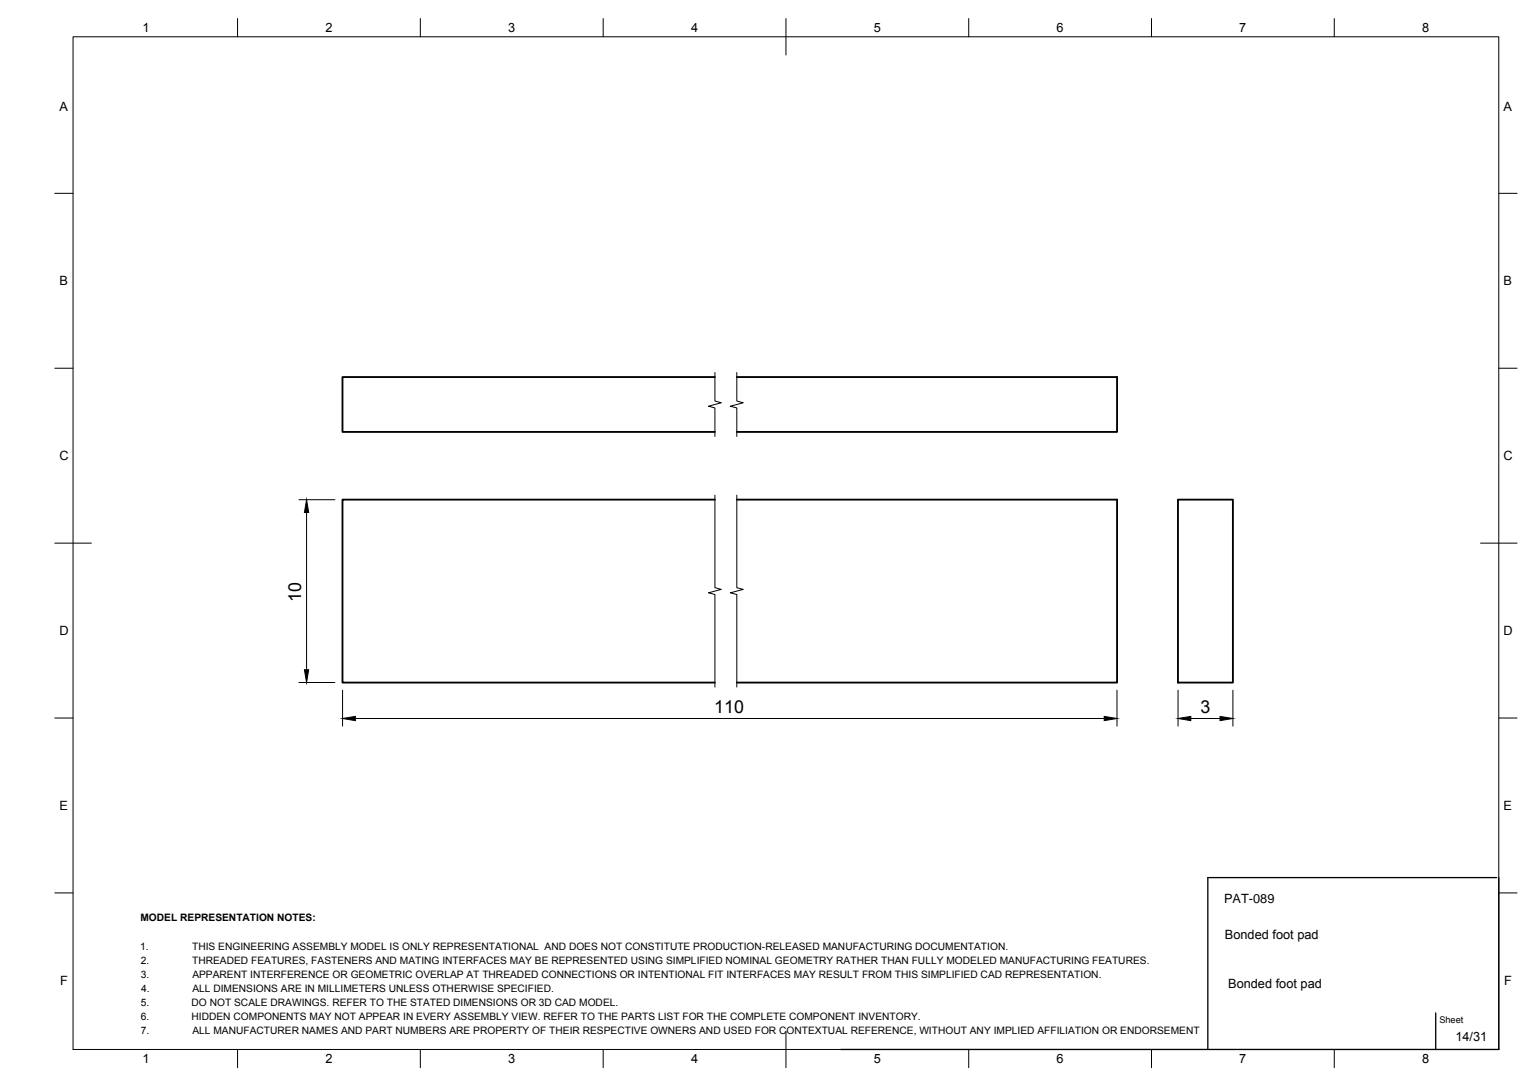
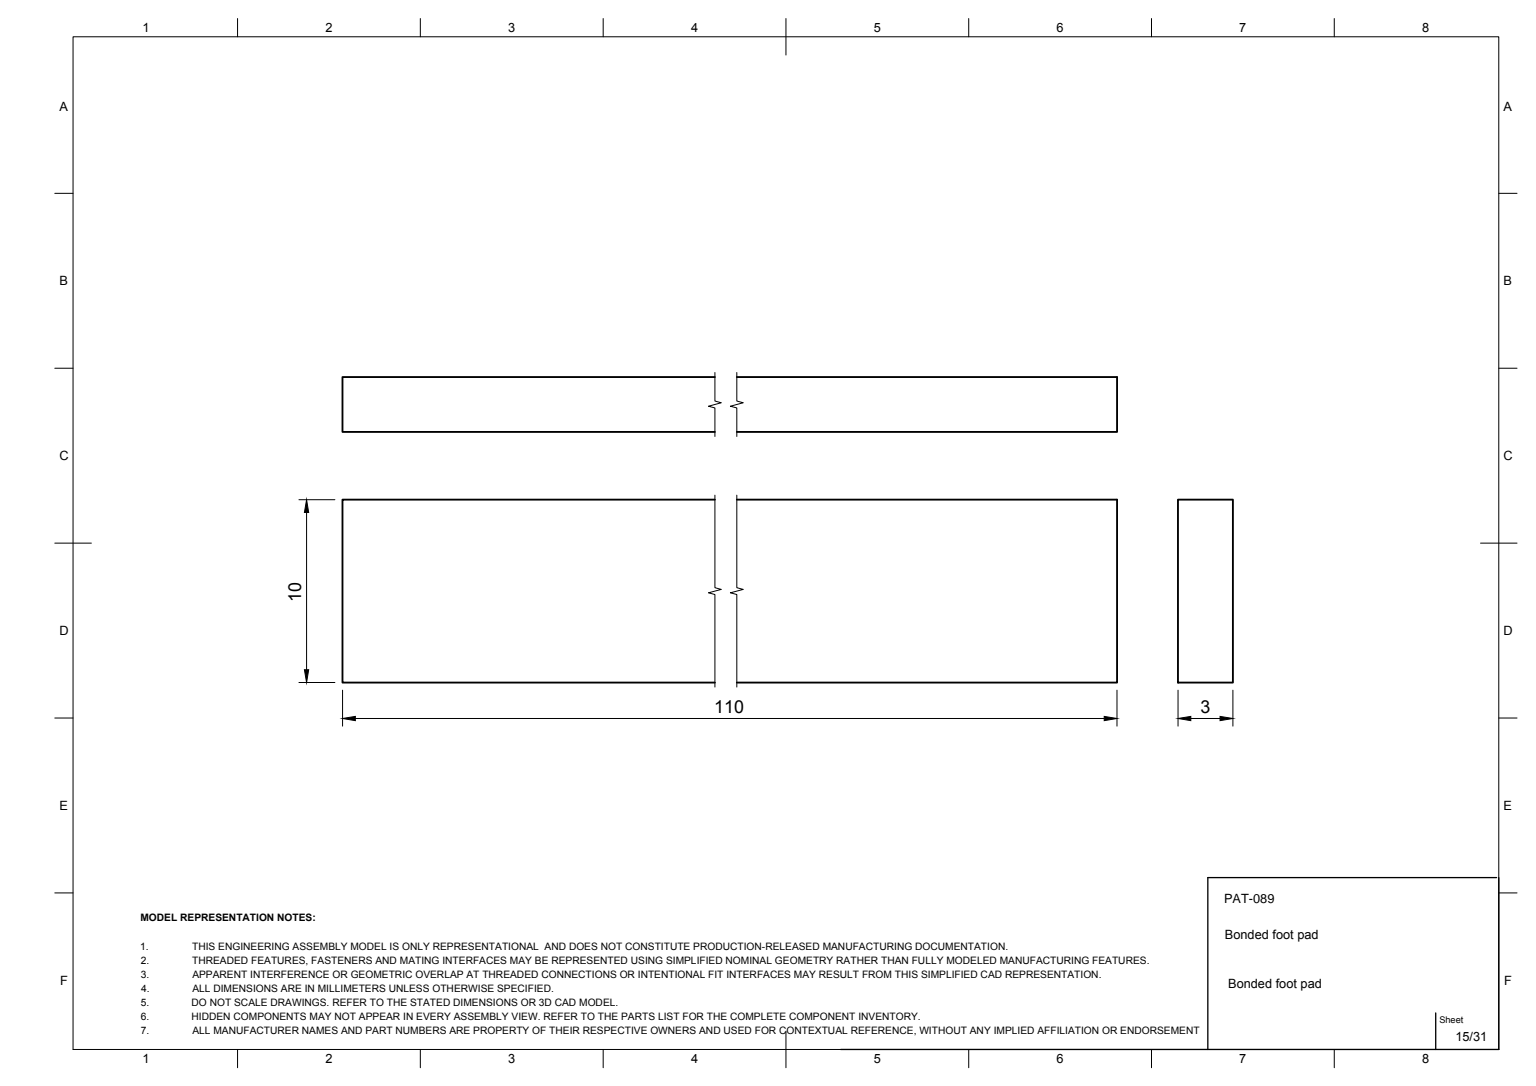
ISO-10303-21;
HEADER;
/* Generated by software containing ST-Developer
 * from STEP Tools, Inc. (www.steptools.com) 
 */

FILE_DESCRIPTION(
/* description */ ('Rotary union on bearing shaft'),
/* implementation_level */ '2;1');

FILE_NAME(
/* name */ 'Bonded foot pad.step',
/* time_stamp */ '2026-10-28T03:24:01-07:00',
/* author */ (''),
/* organization */ (''),
/* preprocessor_version */ 'ST-DEVELOPER v20.2',
/* originating_system */ 'Autodesk Translation Framework v15.17.0.0',
/* authorisation */ '');

FILE_SCHEMA (('AUTOMOTIVE_DESIGN { 1 0 10303 214 3 1 1 }'));
ENDSEC;

DATA;
#10=MECHANICAL_DESIGN_GEOMETRIC_PRESENTATION_REPRESENTATION('',(#322),#9448);
#268=SHAPE_REPRESENTATION_RELATIONSHIP('SRR','None',#9568,#295);
#295=ADVANCED_BREP_SHAPE_REPRESENTATION('',(#357),#9428);
#322=STYLED_ITEM('',(#9771),#357);
#357=MANIFOLD_SOLID_BREP('Body1',#4877);
#538=PLANE('',#5414);
#539=PLANE('',#5415);
#540=PLANE('',#5416);
#541=PLANE('',#5417);
#542=PLANE('',#5418);
#543=PLANE('',#5419);
#755=FACE_OUTER_BOUND('',#1118,.T.);
#756=FACE_OUTER_BOUND('',#1119,.T.);
#757=FACE_OUTER_BOUND('',#1120,.T.);
#758=FACE_OUTER_BOUND('',#1121,.T.);
#759=FACE_OUTER_BOUND('',#1122,.T.);
#760=FACE_OUTER_BOUND('',#1123,.T.);
#1118=EDGE_LOOP('',(#3675,#3676,#3677,#3678));
#1119=EDGE_LOOP('',(#3679,#3680,#3681,#3682));
#1120=EDGE_LOOP('',(#3683,#3684,#3685,#3686));
#1121=EDGE_LOOP('',(#3687,#3688,#3689,#3690));
#1122=EDGE_LOOP('',(#3691,#3692,#3693,#3694));
#1123=EDGE_LOOP('',(#3695,#3696,#3697,#3698));
#1458=LINE('',#7978,#1778);
#1459=LINE('',#7980,#1779);
#1460=LINE('',#7982,#1780);
#1461=LINE('',#7983,#1781);
#1462=LINE('',#7986,#1782);
#1463=LINE('',#7988,#1783);
#1464=LINE('',#7989,#1784);
#1465=LINE('',#7992,#1785);
#1466=LINE('',#7994,#1786);
#1467=LINE('',#7995,#1787);
#1468=LINE('',#7997,#1788);
#1469=LINE('',#7998,#1789);
#1778=VECTOR('',#6347,1.);
#1779=VECTOR('',#6348,1.);
#1780=VECTOR('',#6349,1.);
#1781=VECTOR('',#6350,1.);
#1782=VECTOR('',#6353,1.);
#1783=VECTOR('',#6354,1.);
#1784=VECTOR('',#6355,1.);
#1785=VECTOR('',#6358,1.);
#1786=VECTOR('',#6359,1.);
#1787=VECTOR('',#6360,1.);
#1788=VECTOR('',#6363,1.);
#1789=VECTOR('',#6364,1.);
#2388=VERTEX_POINT('',#7976);
#2389=VERTEX_POINT('',#7977);
#2390=VERTEX_POINT('',#7979);
#2391=VERTEX_POINT('',#7981);
#2392=VERTEX_POINT('',#7985);
#2393=VERTEX_POINT('',#7987);
#2394=VERTEX_POINT('',#7991);
#2395=VERTEX_POINT('',#7993);
#2865=EDGE_CURVE('',#2388,#2389,#1458,.T.);
#2866=EDGE_CURVE('',#2389,#2390,#1459,.T.);
#2867=EDGE_CURVE('',#2391,#2390,#1460,.T.);
#2868=EDGE_CURVE('',#2388,#2391,#1461,.T.);
#2869=EDGE_CURVE('',#2392,#2388,#1462,.T.);
#2870=EDGE_CURVE('',#2393,#2391,#1463,.T.);
#2871=EDGE_CURVE('',#2392,#2393,#1464,.T.);
#2872=EDGE_CURVE('',#2394,#2392,#1465,.T.);
#2873=EDGE_CURVE('',#2395,#2393,#1466,.T.);
#2874=EDGE_CURVE('',#2394,#2395,#1467,.T.);
#2875=EDGE_CURVE('',#2389,#2394,#1468,.T.);
#2876=EDGE_CURVE('',#2390,#2395,#1469,.T.);
#3675=ORIENTED_EDGE('',*,*,#2865,.T.);
#3676=ORIENTED_EDGE('',*,*,#2866,.T.);
#3677=ORIENTED_EDGE('',*,*,#2867,.F.);
#3678=ORIENTED_EDGE('',*,*,#2868,.F.);
#3679=ORIENTED_EDGE('',*,*,#2869,.T.);
#3680=ORIENTED_EDGE('',*,*,#2868,.T.);
#3681=ORIENTED_EDGE('',*,*,#2870,.F.);
#3682=ORIENTED_EDGE('',*,*,#2871,.F.);
#3683=ORIENTED_EDGE('',*,*,#2872,.T.);
#3684=ORIENTED_EDGE('',*,*,#2871,.T.);
#3685=ORIENTED_EDGE('',*,*,#2873,.F.);
#3686=ORIENTED_EDGE('',*,*,#2874,.F.);
#3687=ORIENTED_EDGE('',*,*,#2875,.T.);
#3688=ORIENTED_EDGE('',*,*,#2874,.T.);
#3689=ORIENTED_EDGE('',*,*,#2876,.F.);
#3690=ORIENTED_EDGE('',*,*,#2866,.F.);
#3691=ORIENTED_EDGE('',*,*,#2876,.T.);
#3692=ORIENTED_EDGE('',*,*,#2873,.T.);
#3693=ORIENTED_EDGE('',*,*,#2870,.T.);
#3694=ORIENTED_EDGE('',*,*,#2867,.T.);
#3695=ORIENTED_EDGE('',*,*,#2875,.F.);
#3696=ORIENTED_EDGE('',*,*,#2865,.F.);
#3697=ORIENTED_EDGE('',*,*,#2869,.F.);
#3698=ORIENTED_EDGE('',*,*,#2872,.F.);
#4668=ADVANCED_FACE('',(#755),#538,.T.);
#4669=ADVANCED_FACE('',(#756),#539,.T.);
#4670=ADVANCED_FACE('',(#757),#540,.T.);
#4671=ADVANCED_FACE('',(#758),#541,.T.);
#4672=ADVANCED_FACE('',(#759),#542,.T.);
#4673=ADVANCED_FACE('',(#760),#543,.F.);
#4877=CLOSED_SHELL('',(#4668,#4669,#4670,#4671,#4672,#4673));
#5413=AXIS2_PLACEMENT_3D('',#7974,#6343,#6344);
#5414=AXIS2_PLACEMENT_3D('',#7975,#6345,#6346);
#5415=AXIS2_PLACEMENT_3D('',#7984,#6351,#6352);
#5416=AXIS2_PLACEMENT_3D('',#7990,#6356,#6357);
#5417=AXIS2_PLACEMENT_3D('',#7996,#6361,#6362);
#5418=AXIS2_PLACEMENT_3D('',#7999,#6365,#6366);
#5419=AXIS2_PLACEMENT_3D('',#8000,#6367,#6368);
#6343=DIRECTION('axis',(0.,0.,1.));
#6344=DIRECTION('refdir',(1.,0.,0.));
#6345=DIRECTION('center_axis',(0.,1.,0.));
#6346=DIRECTION('ref_axis',(-1.,0.,0.));
#6347=DIRECTION('',(-1.,0.,0.));
#6348=DIRECTION('',(0.,0.,1.));
#6349=DIRECTION('',(-1.,0.,0.));
#6350=DIRECTION('',(0.,0.,1.));
#6351=DIRECTION('center_axis',(1.,0.,0.));
#6352=DIRECTION('ref_axis',(0.,1.,0.));
#6353=DIRECTION('',(0.,1.,0.));
#6354=DIRECTION('',(0.,1.,0.));
#6355=DIRECTION('',(0.,0.,1.));
#6356=DIRECTION('center_axis',(0.,-1.,0.));
#6357=DIRECTION('ref_axis',(1.,0.,0.));
#6358=DIRECTION('',(1.,0.,0.));
#6359=DIRECTION('',(1.,0.,0.));
#6360=DIRECTION('',(0.,0.,1.));
#6361=DIRECTION('center_axis',(-1.,0.,0.));
#6362=DIRECTION('ref_axis',(0.,-1.,0.));
#6363=DIRECTION('',(0.,-1.,0.));
#6364=DIRECTION('',(0.,-1.,0.));
#6365=DIRECTION('center_axis',(0.,0.,1.));
#6366=DIRECTION('ref_axis',(1.,0.,0.));
#6367=DIRECTION('center_axis',(0.,0.,1.));
#6368=DIRECTION('ref_axis',(1.,0.,0.));
#7974=CARTESIAN_POINT('',(0.,0.,0.));
#7975=CARTESIAN_POINT('Origin',(5.5,0.,-0.3));
#7976=CARTESIAN_POINT('',(5.5,0.,-0.3));
#7977=CARTESIAN_POINT('',(-5.5,0.,-0.3));
#7978=CARTESIAN_POINT('',(5.5,0.,-0.3));
#7979=CARTESIAN_POINT('',(-5.5,0.,0.));
#7980=CARTESIAN_POINT('',(-5.5,0.,-0.3));
#7981=CARTESIAN_POINT('',(5.5,0.,0.));
#7982=CARTESIAN_POINT('',(5.5,0.,0.));
#7983=CARTESIAN_POINT('',(5.5,0.,-0.3));
#7984=CARTESIAN_POINT('Origin',(5.5,-1.,-0.3));
#7985=CARTESIAN_POINT('',(5.5,-1.,-0.3));
#7986=CARTESIAN_POINT('',(5.5,-1.,-0.3));
#7987=CARTESIAN_POINT('',(5.5,-1.,0.));
#7988=CARTESIAN_POINT('',(5.5,-1.,0.));
#7989=CARTESIAN_POINT('',(5.5,-1.,-0.3));
#7990=CARTESIAN_POINT('Origin',(-5.5,-1.,-0.3));
#7991=CARTESIAN_POINT('',(-5.5,-1.,-0.3));
#7992=CARTESIAN_POINT('',(-5.5,-1.,-0.3));
#7993=CARTESIAN_POINT('',(-5.5,-1.,0.));
#7994=CARTESIAN_POINT('',(-5.5,-1.,0.));
#7995=CARTESIAN_POINT('',(-5.5,-1.,-0.3));
#7996=CARTESIAN_POINT('Origin',(-5.5,0.,-0.3));
#7997=CARTESIAN_POINT('',(-5.5,0.,-0.3));
#7998=CARTESIAN_POINT('',(-5.5,0.,0.));
#7999=CARTESIAN_POINT('Origin',(0.,-0.5,0.));
#8000=CARTESIAN_POINT('Origin',(0.,-0.5,-0.3));
#9396=UNCERTAINTY_MEASURE_WITH_UNIT(LENGTH_MEASURE(0.001),#9449,
'DISTANCE_ACCURACY_VALUE',
'Maximum model space distance between geometric entities at asserted c
onnectivities');
#9416=UNCERTAINTY_MEASURE_WITH_UNIT(LENGTH_MEASURE(0.001),#9449,
'DISTANCE_ACCURACY_VALUE',
'Maximum model space distance between geometric entities at asserted c
onnectivities');
#9428=(
GEOMETRIC_REPRESENTATION_CONTEXT(3)
GLOBAL_UNCERTAINTY_ASSIGNED_CONTEXT((#9396))
GLOBAL_UNIT_ASSIGNED_CONTEXT((#9449,#9451,#9452))
REPRESENTATION_CONTEXT('','3D')
);
#9448=(
GEOMETRIC_REPRESENTATION_CONTEXT(3)
GLOBAL_UNCERTAINTY_ASSIGNED_CONTEXT((#9416))
GLOBAL_UNIT_ASSIGNED_CONTEXT((#9449,#9451,#9452))
REPRESENTATION_CONTEXT('','3D')
);
#9449=(
LENGTH_UNIT()
NAMED_UNIT(*)
SI_UNIT(.CENTI.,.METRE.)
);
#9451=(
NAMED_UNIT(*)
PLANE_ANGLE_UNIT()
SI_UNIT($,.RADIAN.)
);
#9452=(
NAMED_UNIT(*)
SI_UNIT($,.STERADIAN.)
SOLID_ANGLE_UNIT()
);
#9464=SHAPE_DEFINITION_REPRESENTATION(#9495,#9568);
#9495=PRODUCT_DEFINITION_SHAPE('',$,#9600);
#9568=SHAPE_REPRESENTATION('',(#5413),#9428);
#9588=PRODUCT_DEFINITION_CONTEXT('part definition',#9683,'design');
#9600=PRODUCT_DEFINITION('Bonded foot pad','Bonded foot pad',#9631,#9588);
#9631=PRODUCT_DEFINITION_FORMATION('',$,#9696);
#9683=APPLICATION_CONTEXT(
'Core Data for Automotive Mechanical Design Process');
#9684=PRODUCT_CONTEXT('part definition',#9683,'mechanical');
#9696=PRODUCT('Bonded foot pad','Bonded foot pad','Bonded foot pad',(#9684));
#9765=COLOUR_RGB('Sky Blue',0.24,0.69,0.87);
#9766=FILL_AREA_STYLE_COLOUR('',#9765);
#9767=FILL_AREA_STYLE('',(#9766));
#9768=SURFACE_STYLE_FILL_AREA(#9767);
#9769=SURFACE_SIDE_STYLE('',(#9768));
#9770=SURFACE_STYLE_USAGE(.BOTH.,#9769);
#9771=PRESENTATION_STYLE_ASSIGNMENT((#9770));
ENDSEC;
END-ISO-10303-21;
